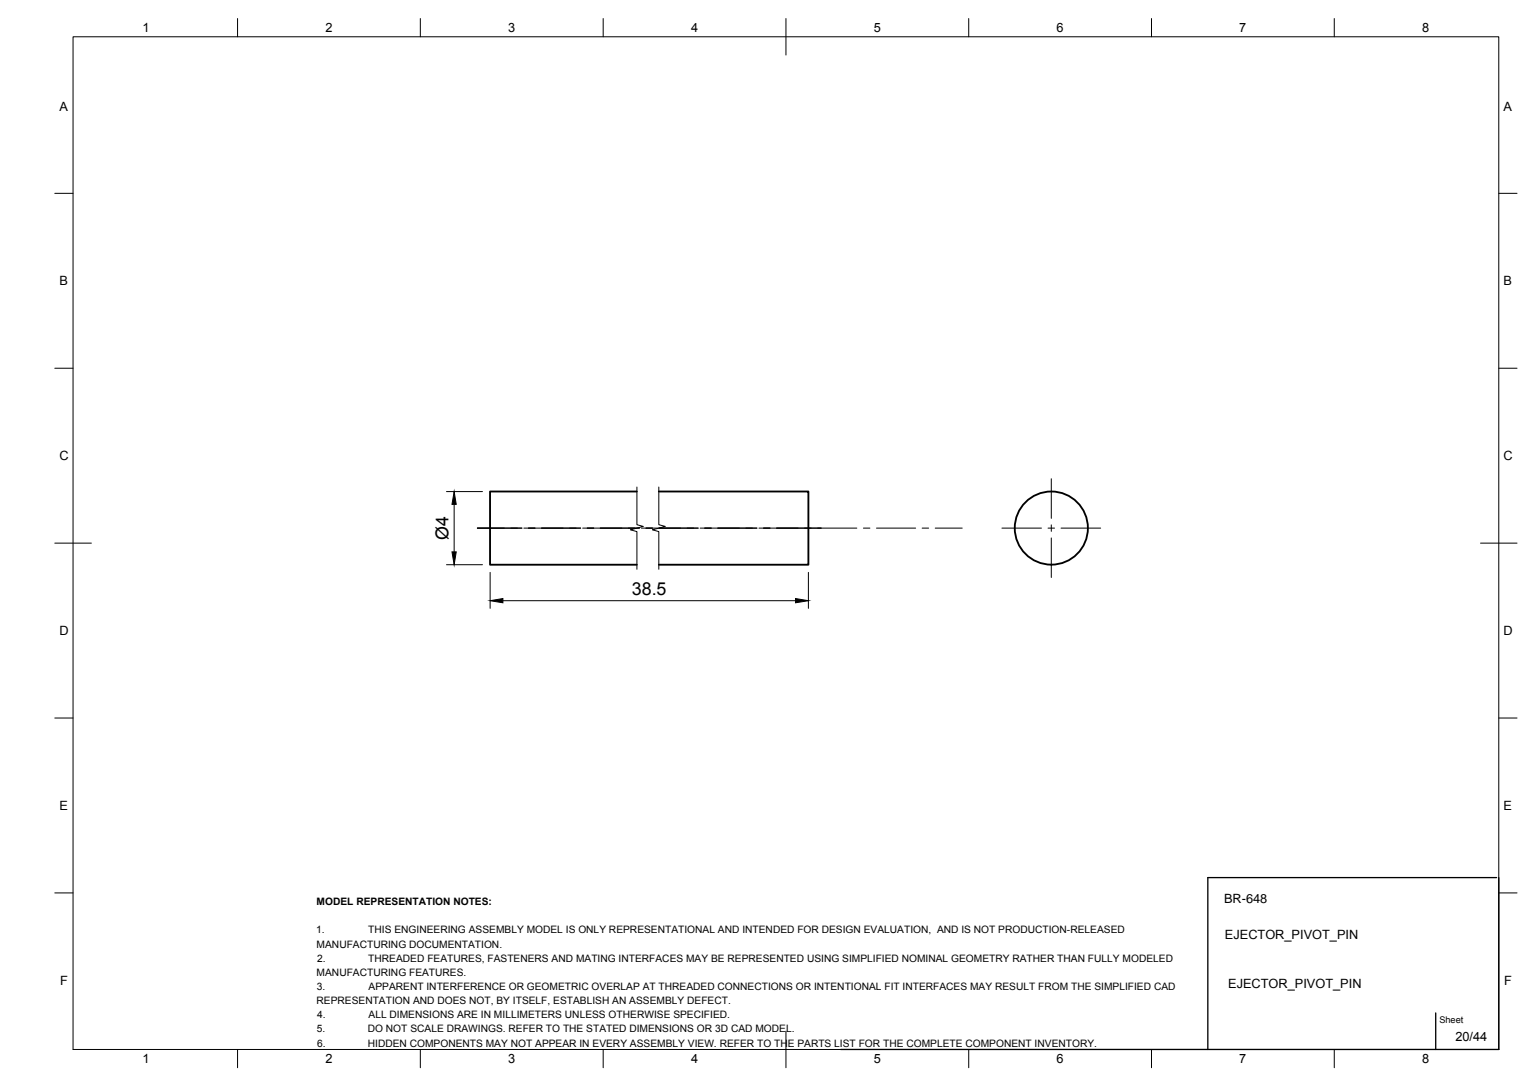
ISO-10303-21;
HEADER;
FILE_DESCRIPTION((''),'2;1');
FILE_NAME('EJECTOR_PIVOT_PIN.step','2026-10-01T22:05:39-07:00',(''),(''),'','','');
FILE_SCHEMA (('AUTOMOTIVE_DESIGN { 1 0 10303 214 3 1 1 }'));
ENDSEC;
DATA;
#10=MECHANICAL_DESIGN_GEOMETRIC_PRESENTATION_REPRESENTATION('',(#620),#24628);
#536=SHAPE_REPRESENTATION_RELATIONSHIP('SRR','None',#24808,#578) ;
#578=ADVANCED_BREP_SHAPE_REPRESENTATION('',(#660),#24598) ;
#620=STYLED_ITEM('',(#25030),#660) ;
#660=MANIFOLD_SOLID_BREP('EJECTOR_PIVOT_PIN',#13131) ;
#1355=LINE('',#21205,#2191) ;
#2191=VECTOR('',#16952,0.2) ;
#2811=CYLINDRICAL_SURFACE('',#14254,0.2) ;
#3241=FACE_OUTER_BOUND('',#4179,.T.) ;
#3242=FACE_OUTER_BOUND('',#4180,.T.) ;
#3243=FACE_OUTER_BOUND('',#4181,.T.) ;
#4179=EDGE_LOOP('',(#9795,#9796,#9797,#9798)) ;
#4180=EDGE_LOOP('',(#9799)) ;
#4181=EDGE_LOOP('',(#9800)) ;
#5046=CIRCLE('',#14255,0.2) ;
#5047=CIRCLE('',#14256,0.2) ;
#5973=VERTEX_POINT('',#21202) ;
#5974=VERTEX_POINT('',#21204) ;
#7387=EDGE_CURVE('',#5973,#5973,#5046,.T.) ;
#7388=EDGE_CURVE('',#5973,#5974,#1355,.T.) ;
#7389=EDGE_CURVE('',#5974,#5974,#5047,.T.) ;
#9795=ORIENTED_EDGE('',*,*,#7387,.F.) ;
#9796=ORIENTED_EDGE('',*,*,#7388,.T.) ;
#9797=ORIENTED_EDGE('',*,*,#7389,.F.) ;
#9798=ORIENTED_EDGE('',*,*,#7388,.F.) ;
#9799=ORIENTED_EDGE('',*,*,#7389,.T.) ;
#9800=ORIENTED_EDGE('',*,*,#7387,.T.) ;
#12146=PLANE('',#14257) ;
#12147=PLANE('',#14258) ;
#12636=ADVANCED_FACE('',(#3241),#2811,.T.) ;
#12637=ADVANCED_FACE('',(#3242),#12146,.T.) ;
#12638=ADVANCED_FACE('',(#3243),#12147,.T.) ;
#13131=CLOSED_SHELL('',(#12636,#12637,#12638)) ;
#14253=AXIS2_PLACEMENT_3D('',#21200,#16946,#16947) ;
#14254=AXIS2_PLACEMENT_3D('',#21201,#16948,#16949) ;
#14255=AXIS2_PLACEMENT_3D('',#21203,#16950,#16951) ;
#14256=AXIS2_PLACEMENT_3D('',#21206,#16953,#16954) ;
#14257=AXIS2_PLACEMENT_3D('',#21207,#16955,#16956) ;
#14258=AXIS2_PLACEMENT_3D('',#21208,#16957,#16958) ;
#16946=DIRECTION('axis',(0.,0.,1.)) ;
#16947=DIRECTION('refdir',(1.,0.,0.)) ;
#16948=DIRECTION('center_axis',(0.,1.,0.)) ;
#16949=DIRECTION('ref_axis',(1.,0.,0.)) ;
#16950=DIRECTION('center_axis',(0.,1.,0.)) ;
#16951=DIRECTION('ref_axis',(1.,0.,0.)) ;
#16952=DIRECTION('',(0.,-1.,0.)) ;
#16953=DIRECTION('center_axis',(0.,-1.,0.)) ;
#16954=DIRECTION('ref_axis',(1.,0.,0.)) ;
#16955=DIRECTION('center_axis',(0.,-1.,0.)) ;
#16956=DIRECTION('ref_axis',(-1.,0.,0.)) ;
#16957=DIRECTION('center_axis',(0.,1.,0.)) ;
#16958=DIRECTION('ref_axis',(1.,0.,0.)) ;
#21200=CARTESIAN_POINT('',(0.,0.,0.)) ;
#21201=CARTESIAN_POINT('Origin',(-6.1946255125913,1.975,8.84684207832111)) ;
#21202=CARTESIAN_POINT('',(-6.3946255125913,3.9,8.84684207832111)) ;
#21203=CARTESIAN_POINT('Origin',(-6.1946255125913,3.9,8.84684207832111)) ;
#21204=CARTESIAN_POINT('',(-6.3946255125913,0.05,8.84684207832111)) ;
#21205=CARTESIAN_POINT('',(-6.3946255125913,1.975,8.84684207832111)) ;
#21206=CARTESIAN_POINT('Origin',(-6.1946255125913,0.0499999999999998,8.84684207832111)) ;
#21207=CARTESIAN_POINT('Origin',(-6.1946255125913,0.0499999999999998,8.84684207832111)) ;
#21208=CARTESIAN_POINT('Origin',(-6.1946255125913,3.9,8.84684207832111)) ;
#24550=UNCERTAINTY_MEASURE_WITH_UNIT(LENGTH_MEASURE(0.001),#24629,
'DISTANCE_ACCURACY_VALUE',
'Maximum model space distance between geometric entities at asserted c
onnectivities') ;
#24580=UNCERTAINTY_MEASURE_WITH_UNIT(LENGTH_MEASURE(0.001),#24629,
'DISTANCE_ACCURACY_VALUE',
'Maximum model space distance between geometric entities at asserted c
onnectivities') ;
#24598=(
GEOMETRIC_REPRESENTATION_CONTEXT(3)
GLOBAL_UNCERTAINTY_ASSIGNED_CONTEXT((#24550))
GLOBAL_UNIT_ASSIGNED_CONTEXT((#24629,#24631,#24632))
REPRESENTATION_CONTEXT('','3D')
) ;
#24628=(
GEOMETRIC_REPRESENTATION_CONTEXT(3)
GLOBAL_UNCERTAINTY_ASSIGNED_CONTEXT((#24580))
GLOBAL_UNIT_ASSIGNED_CONTEXT((#24629,#24631,#24632))
REPRESENTATION_CONTEXT('','3D')
) ;
#24629=(
LENGTH_UNIT()
NAMED_UNIT(*)
SI_UNIT(.CENTI.,.METRE.)
) ;
#24631=(
NAMED_UNIT(*)
PLANE_ANGLE_UNIT()
SI_UNIT($,.RADIAN.)
) ;
#24632=(
NAMED_UNIT(*)
SI_UNIT($,.STERADIAN.)
SOLID_ANGLE_UNIT()
) ;
#24650=SHAPE_DEFINITION_REPRESENTATION(#24697,#24808) ;
#24697=PRODUCT_DEFINITION_SHAPE('',$,#24856) ;
#24808=SHAPE_REPRESENTATION('',(#14253),#24598) ;
#24838=PRODUCT_DEFINITION_CONTEXT('part definition',#24981,'design') ;
#24856=PRODUCT_DEFINITION('EJECTOR_PIVOT_PIN','EJECTOR_PIVOT_PIN',
#24903,#24838) ;
#24903=PRODUCT_DEFINITION_FORMATION('',$,#25000) ;
#24981=APPLICATION_CONTEXT(
'Core Data for Automotive Mechanical Design Process') ;
#24982=PRODUCT_CONTEXT('part definition',#24981,'mechanical') ;
#25000=PRODUCT('EJECTOR_PIVOT_PIN','EJECTOR_PIVOT_PIN',$,(#24982)) ;
#25030=PRESENTATION_STYLE_ASSIGNMENT((#25040)) ;
#25040=SURFACE_STYLE_USAGE(.BOTH.,#25050) ;
#25050=SURFACE_SIDE_STYLE('',(#25060)) ;
#25060=SURFACE_STYLE_FILL_AREA(#25070) ;
#25070=FILL_AREA_STYLE('Steel - Satin',(#25080)) ;
#25080=FILL_AREA_STYLE_COLOUR('Steel - Satin',#25090) ;
#25090=COLOUR_RGB('Steel - Satin', 0.66274510, 0.83137255, 0.94901961) ;
ENDSEC;
END-ISO-10303-21;
